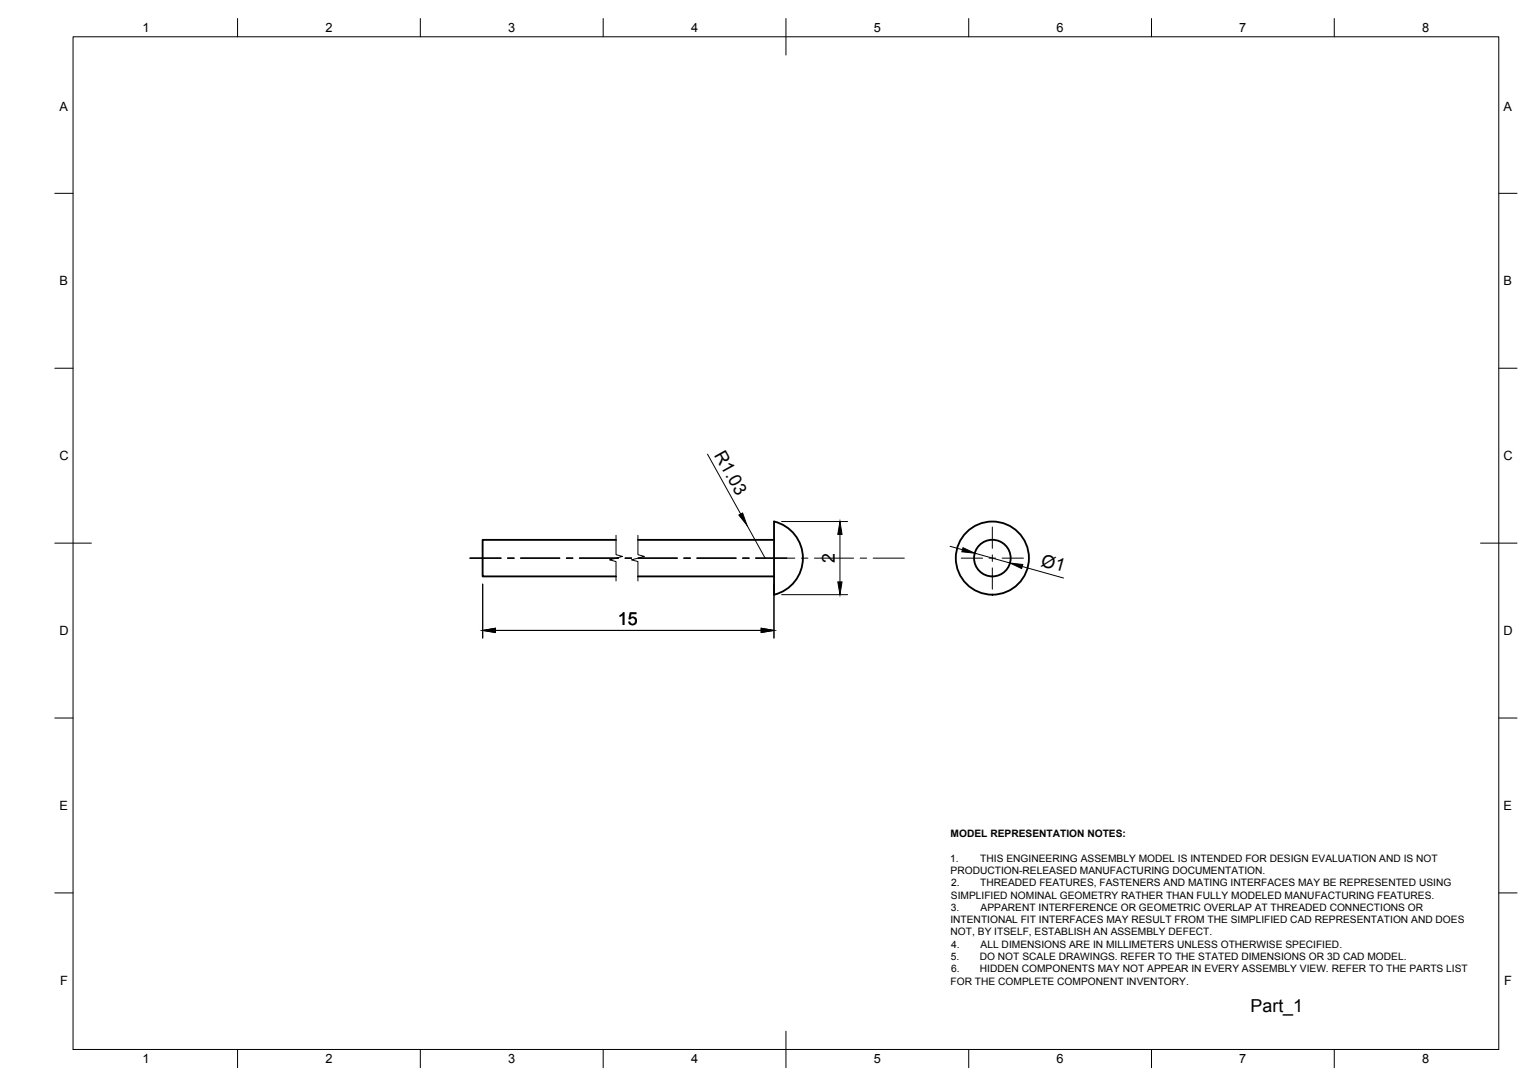
ISO-10303-21;
HEADER;
/* Generated by software containing ST-Developer
 * from STEP Tools, Inc. (www.steptools.com) 
 */

FILE_DESCRIPTION(
/* description */ ('STEP AP242 Edition 2'),
/* implementation_level */ '2;1');

FILE_NAME(
/* name */ 'Part_1.step',
/* time_stamp */ '2026-10-06T10:11:12-07:00',
/* author */ (''),
/* organization */ (''),
/* preprocessor_version */ 'ST-DEVELOPER v20.2',
/* originating_system */ 'Autodesk Translation Framework v15.15.0.0',
/* authorisation */ '');

FILE_SCHEMA (('AUTOMOTIVE_DESIGN { 1 0 10303 214 3 1 1 }'));
ENDSEC;

DATA;
#10=MECHANICAL_DESIGN_GEOMETRIC_PRESENTATION_REPRESENTATION('',(#1800),#54580);
#170=SPHERICAL_SURFACE('',#19578,0.00102870127000254);
#1756=SHAPE_REPRESENTATION_RELATIONSHIP('SRR','None',#54643,#1770);
#1770=ADVANCED_BREP_SHAPE_REPRESENTATION('',(#1814),#54579);
#1800=STYLED_ITEM('',(#54716),#1814);
#1814=MANIFOLD_SOLID_BREP('Body1',#17679);
#2407=LINE('',#54532,#3000);
#3000=VECTOR('',#23693,0.0005);
#3476=CYLINDRICAL_SURFACE('',#19583,0.0005);
#3543=FACE_BOUND('',#5622,.T.);
#4546=FACE_OUTER_BOUND('',#5618,.T.);
#4547=FACE_OUTER_BOUND('',#5619,.T.);
#4548=FACE_OUTER_BOUND('',#5620,.T.);
#4549=FACE_OUTER_BOUND('',#5621,.T.);
#5618=EDGE_LOOP('',(#16545,#16546,#16547));
#5619=EDGE_LOOP('',(#16548));
#5620=EDGE_LOOP('',(#16549,#16550,#16551,#16552));
#5621=EDGE_LOOP('',(#16553));
#5622=EDGE_LOOP('',(#16554));
#6522=CIRCLE('',#19579,0.001);
#6523=CIRCLE('',#19580,0.00102870127000254);
#6524=CIRCLE('',#19582,0.0005);
#6525=CIRCLE('',#19584,0.0005);
#8322=VERTEX_POINT('',#54522);
#8323=VERTEX_POINT('',#54524);
#8324=VERTEX_POINT('',#54527);
#8325=VERTEX_POINT('',#54530);
#11064=EDGE_CURVE('',#8322,#8322,#6522,.T.);
#11065=EDGE_CURVE('',#8323,#8322,#6523,.T.);
#11066=EDGE_CURVE('',#8324,#8324,#6524,.T.);
#11067=EDGE_CURVE('',#8325,#8325,#6525,.T.);
#11068=EDGE_CURVE('',#8325,#8324,#2407,.T.);
#16545=ORIENTED_EDGE('',*,*,#11064,.T.);
#16546=ORIENTED_EDGE('',*,*,#11065,.F.);
#16547=ORIENTED_EDGE('',*,*,#11065,.T.);
#16548=ORIENTED_EDGE('',*,*,#11066,.F.);
#16549=ORIENTED_EDGE('',*,*,#11067,.F.);
#16550=ORIENTED_EDGE('',*,*,#11068,.T.);
#16551=ORIENTED_EDGE('',*,*,#11066,.T.);
#16552=ORIENTED_EDGE('',*,*,#11068,.F.);
#16553=ORIENTED_EDGE('',*,*,#11064,.F.);
#16554=ORIENTED_EDGE('',*,*,#11067,.T.);
#16658=PLANE('',#19581);
#16659=PLANE('',#19585);
#17662=ADVANCED_FACE('',(#4546),#170,.T.);
#17663=ADVANCED_FACE('',(#4547),#16658,.F.);
#17664=ADVANCED_FACE('',(#4548),#3476,.T.);
#17665=ADVANCED_FACE('',(#4549,#3543),#16659,.F.);
#17679=CLOSED_SHELL('',(#17662,#17663,#17664,#17665));
#19577=AXIS2_PLACEMENT_3D('',#54520,#23677,#23678);
#19578=AXIS2_PLACEMENT_3D('',#54521,#23679,#23680);
#19579=AXIS2_PLACEMENT_3D('',#54523,#23681,#23682);
#19580=AXIS2_PLACEMENT_3D('',#54525,#23683,#23684);
#19581=AXIS2_PLACEMENT_3D('',#54526,#23685,#23686);
#19582=AXIS2_PLACEMENT_3D('',#54528,#23687,#23688);
#19583=AXIS2_PLACEMENT_3D('',#54529,#23689,#23690);
#19584=AXIS2_PLACEMENT_3D('',#54531,#23691,#23692);
#19585=AXIS2_PLACEMENT_3D('',#54533,#23694,#23695);
#23677=DIRECTION('axis',(0.,0.,1.));
#23678=DIRECTION('refdir',(1.,0.,0.));
#23679=DIRECTION('center_axis',(-6.12323399573677E-17,0.,1.));
#23680=DIRECTION('ref_axis',(-1.,0.,0.));
#23681=DIRECTION('center_axis',(0.,0.,1.));
#23682=DIRECTION('ref_axis',(1.,0.,0.));
#23683=DIRECTION('center_axis',(-1.22464679914735E-16,1.,0.));
#23684=DIRECTION('ref_axis',(1.,1.22464679914735E-16,0.));
#23685=DIRECTION('center_axis',(0.,0.,1.));
#23686=DIRECTION('ref_axis',(1.,0.,0.));
#23687=DIRECTION('center_axis',(0.,0.,1.));
#23688=DIRECTION('ref_axis',(1.,0.,0.));
#23689=DIRECTION('center_axis',(0.,0.,1.));
#23690=DIRECTION('ref_axis',(1.,0.,0.));
#23691=DIRECTION('center_axis',(0.,0.,1.));
#23692=DIRECTION('ref_axis',(1.,0.,0.));
#23693=DIRECTION('',(0.,0.,-1.));
#23694=DIRECTION('center_axis',(0.,0.,1.));
#23695=DIRECTION('ref_axis',(1.,0.,0.));
#54520=CARTESIAN_POINT('',(0.,0.,0.));
#54521=CARTESIAN_POINT('Origin',(0.,0.,-0.00102870127000254));
#54522=CARTESIAN_POINT('',(0.001,0.,-0.0007874));
#54523=CARTESIAN_POINT('Origin',(0.,0.,-0.0007874));
#54524=CARTESIAN_POINT('',(6.29897858793714E-20,7.71402396561493E-36,0.));
#54525=CARTESIAN_POINT('Origin',(0.,0.,-0.00102870127000254));
#54526=CARTESIAN_POINT('Origin',(0.,0.,-0.0157874));
#54527=CARTESIAN_POINT('',(-0.0005,-6.12323399573677E-20,-0.0157874));
#54528=CARTESIAN_POINT('Origin',(0.,0.,-0.0157874));
#54529=CARTESIAN_POINT('Origin',(0.,0.,0.));
#54530=CARTESIAN_POINT('',(-0.0005,-6.12323399573677E-20,-0.0007874));
#54531=CARTESIAN_POINT('Origin',(0.,0.,-0.0007874));
#54532=CARTESIAN_POINT('',(-0.0005,-6.12323399573677E-20,0.));
#54533=CARTESIAN_POINT('Origin',(-0.001,0.,-0.0007874));
#54563=UNCERTAINTY_MEASURE_WITH_UNIT(LENGTH_MEASURE(1.E-5),#54581,
'DISTANCE_ACCURACY_VALUE',
'Maximum model space distance between geometric entities at asserted c
onnectivities');
#54564=UNCERTAINTY_MEASURE_WITH_UNIT(LENGTH_MEASURE(1.E-5),#54581,
'DISTANCE_ACCURACY_VALUE',
'Maximum model space distance between geometric entities at asserted c
onnectivities');
#54579=(
GEOMETRIC_REPRESENTATION_CONTEXT(3)
GLOBAL_UNCERTAINTY_ASSIGNED_CONTEXT((#54563))
GLOBAL_UNIT_ASSIGNED_CONTEXT((#54581,#54582,#54583))
REPRESENTATION_CONTEXT('','3D')
);
#54580=(
GEOMETRIC_REPRESENTATION_CONTEXT(3)
GLOBAL_UNCERTAINTY_ASSIGNED_CONTEXT((#54564))
GLOBAL_UNIT_ASSIGNED_CONTEXT((#54581,#54582,#54583))
REPRESENTATION_CONTEXT('','3D')
);
#54581=(
LENGTH_UNIT()
NAMED_UNIT(*)
SI_UNIT($,.METRE.)
);
#54582=(
NAMED_UNIT(*)
PLANE_ANGLE_UNIT()
SI_UNIT($,.RADIAN.)
);
#54583=(
NAMED_UNIT(*)
SI_UNIT($,.STERADIAN.)
SOLID_ANGLE_UNIT()
);
#54598=SHAPE_DEFINITION_REPRESENTATION(#54613,#54643);
#54613=PRODUCT_DEFINITION_SHAPE('',$,#54659);
#54643=SHAPE_REPRESENTATION('',(#19577),#54579);
#54644=PRODUCT_DEFINITION_CONTEXT('part definition',#54691,'design');
#54659=PRODUCT_DEFINITION('Part_1','Part_1',#54674,#54644);
#54674=PRODUCT_DEFINITION_FORMATION('',$,#54707);
#54691=APPLICATION_CONTEXT(
'Core Data for Automotive Mechanical Design Process');
#54692=PRODUCT_CONTEXT('part definition',#54691,'mechanical');
#54707=PRODUCT('Part_1','Part_1','Part 1',(#54692));
#54716=PRESENTATION_STYLE_ASSIGNMENT((#54726));
#54726=SURFACE_STYLE_USAGE(.BOTH.,#54736);
#54736=SURFACE_SIDE_STYLE('',(#54746));
#54746=SURFACE_STYLE_FILL_AREA(#54756);
#54756=FILL_AREA_STYLE('Opaque(76,76,76)',(#54766));
#54766=FILL_AREA_STYLE_COLOUR('Opaque(76,76,76)',#54776);
#54776=COLOUR_RGB('Opaque(76,76,76)', 0.08235294, 0.09019608, 0.10196078);
ENDSEC;
END-ISO-10303-21;
